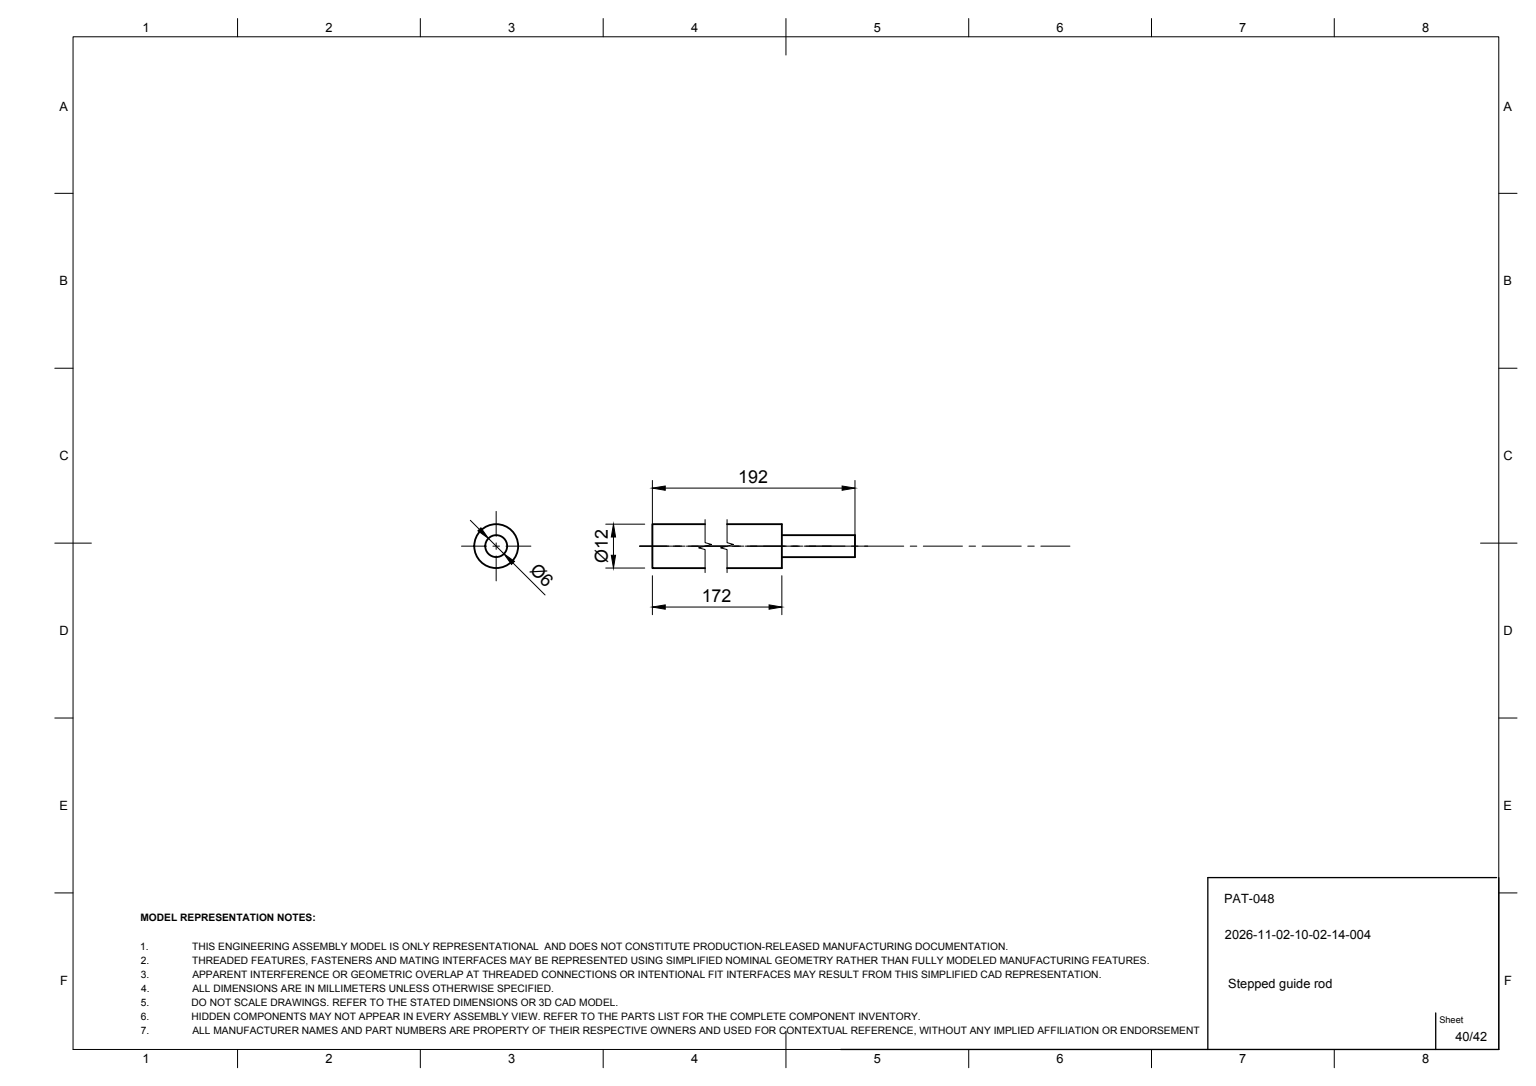
ISO-10303-21;
HEADER;
/* Generated by software containing ST-Developer
 * from STEP Tools, Inc. (www.steptools.com) 
 */

FILE_DESCRIPTION(
/* description */ ('Guided pneumatic stop gate'),
/* implementation_level */ '2;1');

FILE_NAME(
/* name */ 'Stepped guide rod.step',
/* time_stamp */ '2026-10-27T21:43:45-07:00',
/* author */ (''),
/* organization */ (''),
/* preprocessor_version */ 'ST-DEVELOPER v20.2',
/* originating_system */ 'Autodesk Translation Framework v15.17.0.0',
/* authorisation */ '');

FILE_SCHEMA (('AUTOMOTIVE_DESIGN { 1 0 10303 214 3 1 1 }'));
ENDSEC;

DATA;
#10=MECHANICAL_DESIGN_GEOMETRIC_PRESENTATION_REPRESENTATION('',(#572),#14392);
#488=SHAPE_REPRESENTATION_RELATIONSHIP('SRR','None',#14625,#530);
#530=ADVANCED_BREP_SHAPE_REPRESENTATION('',(#610),#14387);
#572=STYLED_ITEM('',(#14891),#610);
#610=MANIFOLD_SOLID_BREP('Body1',#7916);
#812=FACE_BOUND('',#2231,.T.);
#1091=PLANE('',#9299);
#1092=PLANE('',#9303);
#1093=PLANE('',#9304);
#1554=FACE_OUTER_BOUND('',#2226,.T.);
#1555=FACE_OUTER_BOUND('',#2227,.T.);
#1556=FACE_OUTER_BOUND('',#2228,.T.);
#1557=FACE_OUTER_BOUND('',#2229,.T.);
#1558=FACE_OUTER_BOUND('',#2230,.T.);
#2226=EDGE_LOOP('',(#7084,#7085,#7086,#7087));
#2227=EDGE_LOOP('',(#7088));
#2228=EDGE_LOOP('',(#7089,#7090,#7091,#7092));
#2229=EDGE_LOOP('',(#7093));
#2230=EDGE_LOOP('',(#7094));
#2231=EDGE_LOOP('',(#7095));
#2781=LINE('',#14088,#3326);
#2782=LINE('',#14095,#3327);
#3326=VECTOR('',#11712,0.3);
#3327=VECTOR('',#11721,0.6);
#3715=CIRCLE('',#9297,0.3);
#3716=CIRCLE('',#9298,0.3);
#3717=CIRCLE('',#9301,0.6);
#3718=CIRCLE('',#9302,0.6);
#4306=VERTEX_POINT('',#14085);
#4307=VERTEX_POINT('',#14087);
#4308=VERTEX_POINT('',#14092);
#4309=VERTEX_POINT('',#14094);
#5240=EDGE_CURVE('',#4306,#4306,#3715,.T.);
#5241=EDGE_CURVE('',#4306,#4307,#2781,.T.);
#5242=EDGE_CURVE('',#4307,#4307,#3716,.T.);
#5243=EDGE_CURVE('',#4308,#4308,#3717,.T.);
#5244=EDGE_CURVE('',#4308,#4309,#2782,.T.);
#5245=EDGE_CURVE('',#4309,#4309,#3718,.T.);
#7084=ORIENTED_EDGE('',*,*,#5240,.F.);
#7085=ORIENTED_EDGE('',*,*,#5241,.T.);
#7086=ORIENTED_EDGE('',*,*,#5242,.T.);
#7087=ORIENTED_EDGE('',*,*,#5241,.F.);
#7088=ORIENTED_EDGE('',*,*,#5242,.F.);
#7089=ORIENTED_EDGE('',*,*,#5243,.F.);
#7090=ORIENTED_EDGE('',*,*,#5244,.T.);
#7091=ORIENTED_EDGE('',*,*,#5245,.T.);
#7092=ORIENTED_EDGE('',*,*,#5244,.F.);
#7093=ORIENTED_EDGE('',*,*,#5243,.T.);
#7094=ORIENTED_EDGE('',*,*,#5245,.F.);
#7095=ORIENTED_EDGE('',*,*,#5240,.T.);
#7390=CYLINDRICAL_SURFACE('',#9296,0.3);
#7391=CYLINDRICAL_SURFACE('',#9300,0.6);
#7836=ADVANCED_FACE('',(#1554),#7390,.T.);
#7837=ADVANCED_FACE('',(#1555),#1091,.F.);
#7838=ADVANCED_FACE('',(#1556),#7391,.T.);
#7839=ADVANCED_FACE('',(#1557),#1092,.T.);
#7840=ADVANCED_FACE('',(#1558,#812),#1093,.F.);
#7916=CLOSED_SHELL('',(#7836,#7837,#7838,#7839,#7840));
#9295=AXIS2_PLACEMENT_3D('',#14083,#11706,#11707);
#9296=AXIS2_PLACEMENT_3D('',#14084,#11708,#11709);
#9297=AXIS2_PLACEMENT_3D('',#14086,#11710,#11711);
#9298=AXIS2_PLACEMENT_3D('',#14089,#11713,#11714);
#9299=AXIS2_PLACEMENT_3D('',#14090,#11715,#11716);
#9300=AXIS2_PLACEMENT_3D('',#14091,#11717,#11718);
#9301=AXIS2_PLACEMENT_3D('',#14093,#11719,#11720);
#9302=AXIS2_PLACEMENT_3D('',#14096,#11722,#11723);
#9303=AXIS2_PLACEMENT_3D('',#14097,#11724,#11725);
#9304=AXIS2_PLACEMENT_3D('',#14098,#11726,#11727);
#11706=DIRECTION('axis',(0.,0.,1.));
#11707=DIRECTION('refdir',(1.,0.,0.));
#11708=DIRECTION('center_axis',(0.,1.,0.));
#11709=DIRECTION('ref_axis',(1.,0.,0.));
#11710=DIRECTION('center_axis',(0.,1.,0.));
#11711=DIRECTION('ref_axis',(1.,0.,0.));
#11712=DIRECTION('',(0.,-1.,0.));
#11713=DIRECTION('center_axis',(0.,1.,0.));
#11714=DIRECTION('ref_axis',(1.,0.,0.));
#11715=DIRECTION('center_axis',(0.,1.,0.));
#11716=DIRECTION('ref_axis',(1.,0.,0.));
#11717=DIRECTION('center_axis',(0.,1.,0.));
#11718=DIRECTION('ref_axis',(1.,0.,0.));
#11719=DIRECTION('center_axis',(0.,1.,0.));
#11720=DIRECTION('ref_axis',(1.,0.,0.));
#11721=DIRECTION('',(0.,-1.,0.));
#11722=DIRECTION('center_axis',(0.,1.,0.));
#11723=DIRECTION('ref_axis',(1.,0.,0.));
#11724=DIRECTION('center_axis',(0.,1.,0.));
#11725=DIRECTION('ref_axis',(1.,0.,0.));
#11726=DIRECTION('center_axis',(0.,1.,0.));
#11727=DIRECTION('ref_axis',(1.,0.,0.));
#14083=CARTESIAN_POINT('',(0.,0.,0.));
#14084=CARTESIAN_POINT('Origin',(-5.,-9.4,4.5));
#14085=CARTESIAN_POINT('',(-5.3,-7.4,4.5));
#14086=CARTESIAN_POINT('Origin',(-5.,-7.4,4.5));
#14087=CARTESIAN_POINT('',(-5.3,-9.4,4.5));
#14088=CARTESIAN_POINT('',(-5.3,-9.4,4.5));
#14089=CARTESIAN_POINT('Origin',(-5.,-9.4,4.5));
#14090=CARTESIAN_POINT('Origin',(-5.,-9.4,4.5));
#14091=CARTESIAN_POINT('Origin',(-5.,-7.4,4.5));
#14092=CARTESIAN_POINT('',(-5.6,9.8,4.5));
#14093=CARTESIAN_POINT('Origin',(-5.,9.8,4.5));
#14094=CARTESIAN_POINT('',(-5.6,-7.4,4.5));
#14095=CARTESIAN_POINT('',(-5.6,-7.4,4.5));
#14096=CARTESIAN_POINT('Origin',(-5.,-7.4,4.5));
#14097=CARTESIAN_POINT('Origin',(-5.,9.8,4.5));
#14098=CARTESIAN_POINT('Origin',(-5.,-7.4,4.5));
#14339=UNCERTAINTY_MEASURE_WITH_UNIT(LENGTH_MEASURE(0.001),#14393,
'DISTANCE_ACCURACY_VALUE',
'Maximum model space distance between geometric entities at asserted c
onnectivities');
#14344=UNCERTAINTY_MEASURE_WITH_UNIT(LENGTH_MEASURE(0.001),#14393,
'DISTANCE_ACCURACY_VALUE',
'Maximum model space distance between geometric entities at asserted c
onnectivities');
#14387=(
GEOMETRIC_REPRESENTATION_CONTEXT(3)
GLOBAL_UNCERTAINTY_ASSIGNED_CONTEXT((#14339))
GLOBAL_UNIT_ASSIGNED_CONTEXT((#14393,#14395,#14396))
REPRESENTATION_CONTEXT('','3D')
);
#14392=(
GEOMETRIC_REPRESENTATION_CONTEXT(3)
GLOBAL_UNCERTAINTY_ASSIGNED_CONTEXT((#14344))
GLOBAL_UNIT_ASSIGNED_CONTEXT((#14393,#14395,#14396))
REPRESENTATION_CONTEXT('','3D')
);
#14393=(
LENGTH_UNIT()
NAMED_UNIT(*)
SI_UNIT(.CENTI.,.METRE.)
);
#14395=(
NAMED_UNIT(*)
PLANE_ANGLE_UNIT()
SI_UNIT($,.RADIAN.)
);
#14396=(
NAMED_UNIT(*)
SI_UNIT($,.STERADIAN.)
SOLID_ANGLE_UNIT()
);
#14439=SHAPE_DEFINITION_REPRESENTATION(#14558,#14625);
#14558=PRODUCT_DEFINITION_SHAPE('',$,#14673);
#14625=SHAPE_REPRESENTATION('',(#9295),#14387);
#14630=PRODUCT_DEFINITION_CONTEXT('part definition',#14773,'design');
#14673=PRODUCT_DEFINITION('Stepped guide rod','Stepped guide rod',#14720,
#14630);
#14720=PRODUCT_DEFINITION_FORMATION('',$,#14817);
#14773=APPLICATION_CONTEXT(
'Core Data for Automotive Mechanical Design Process');
#14774=PRODUCT_CONTEXT('part definition',#14773,'mechanical');
#14817=PRODUCT('Stepped guide rod','Stepped guide rod',
'Stepped guide rod',(#14774));
#14885=COLOUR_RGB('Grey',0.48,0.52,0.57);
#14886=FILL_AREA_STYLE_COLOUR('',#14885);
#14887=FILL_AREA_STYLE('',(#14886));
#14888=SURFACE_STYLE_FILL_AREA(#14887);
#14889=SURFACE_SIDE_STYLE('',(#14888));
#14890=SURFACE_STYLE_USAGE(.BOTH.,#14889);
#14891=PRESENTATION_STYLE_ASSIGNMENT((#14890));
ENDSEC;
END-ISO-10303-21;
